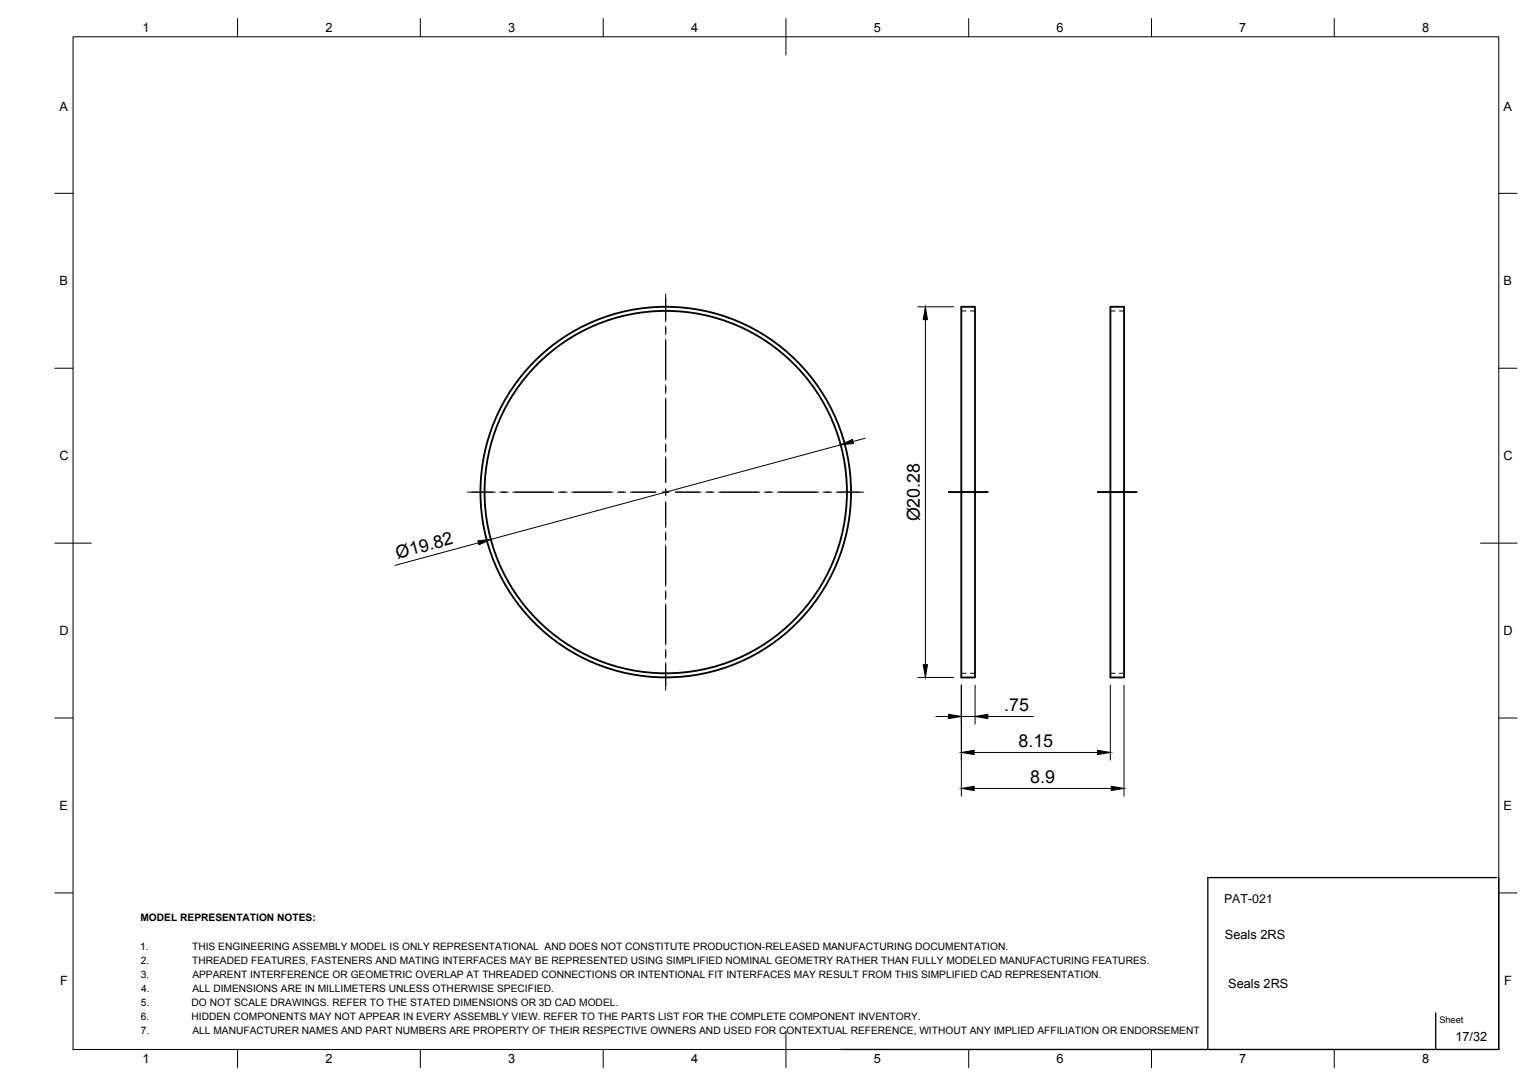
ISO-10303-21;
HEADER;
/* Generated by software containing ST-Developer
 * from STEP Tools, Inc. (www.steptools.com) 
 */

FILE_DESCRIPTION(
/* description */ ('Chain-less indexing wheel (Geneva) drive'),
/* implementation_level */ '2;1');

FILE_NAME(
/* name */ 'Seals 2RS.step',
/* time_stamp */ '2026-10-28T03:25:22-07:00',
/* author */ (''),
/* organization */ (''),
/* preprocessor_version */ 'ST-DEVELOPER v20.2',
/* originating_system */ 'Autodesk Translation Framework v15.17.0.0',
/* authorisation */ '');

FILE_SCHEMA (('AUTOMOTIVE_DESIGN { 1 0 10303 214 3 1 1 }'));
ENDSEC;

DATA;
#10=MECHANICAL_DESIGN_GEOMETRIC_PRESENTATION_REPRESENTATION('',(#321,#322),#10957);
#264=SHAPE_REPRESENTATION_RELATIONSHIP('SRR','None',#11078,#289);
#289=ADVANCED_BREP_SHAPE_REPRESENTATION('',(#353,#354),#10941);
#321=STYLED_ITEM('',(#11287),#353);
#322=STYLED_ITEM('',(#11287),#354);
#353=MANIFOLD_SOLID_BREP('Body1',#5718);
#354=MANIFOLD_SOLID_BREP('Body2',#5719);
#429=FACE_BOUND('',#1216,.T.);
#430=FACE_BOUND('',#1219,.T.);
#431=FACE_BOUND('',#1222,.T.);
#432=FACE_BOUND('',#1225,.T.);
#552=PLANE('',#6383);
#553=PLANE('',#6388);
#554=PLANE('',#6391);
#555=PLANE('',#6396);
#820=FACE_OUTER_BOUND('',#1215,.T.);
#821=FACE_OUTER_BOUND('',#1217,.T.);
#822=FACE_OUTER_BOUND('',#1218,.T.);
#823=FACE_OUTER_BOUND('',#1220,.T.);
#824=FACE_OUTER_BOUND('',#1221,.T.);
#825=FACE_OUTER_BOUND('',#1223,.T.);
#826=FACE_OUTER_BOUND('',#1224,.T.);
#827=FACE_OUTER_BOUND('',#1226,.T.);
#1215=EDGE_LOOP('',(#4487));
#1216=EDGE_LOOP('',(#4488));
#1217=EDGE_LOOP('',(#4489,#4490,#4491,#4492));
#1218=EDGE_LOOP('',(#4493));
#1219=EDGE_LOOP('',(#4494));
#1220=EDGE_LOOP('',(#4495,#4496,#4497,#4498));
#1221=EDGE_LOOP('',(#4499));
#1222=EDGE_LOOP('',(#4500));
#1223=EDGE_LOOP('',(#4501,#4502,#4503,#4504));
#1224=EDGE_LOOP('',(#4505));
#1225=EDGE_LOOP('',(#4506));
#1226=EDGE_LOOP('',(#4507,#4508,#4509,#4510));
#1583=LINE('',#9810,#1957);
#1584=LINE('',#9815,#1958);
#1585=LINE('',#9824,#1959);
#1586=LINE('',#9829,#1960);
#1957=VECTOR('',#7665,1.013815);
#1958=VECTOR('',#7672,0.991185);
#1959=VECTOR('',#7683,1.013815);
#1960=VECTOR('',#7690,0.991185);
#2361=CIRCLE('',#6384,1.013815);
#2362=CIRCLE('',#6385,0.991185);
#2363=CIRCLE('',#6387,1.013815);
#2364=CIRCLE('',#6389,0.991185);
#2365=CIRCLE('',#6392,1.013815);
#2366=CIRCLE('',#6393,0.991185);
#2367=CIRCLE('',#6395,1.013815);
#2368=CIRCLE('',#6397,0.991185);
#2749=VERTEX_POINT('',#9803);
#2750=VERTEX_POINT('',#9805);
#2751=VERTEX_POINT('',#9808);
#2752=VERTEX_POINT('',#9812);
#2753=VERTEX_POINT('',#9817);
#2754=VERTEX_POINT('',#9819);
#2755=VERTEX_POINT('',#9822);
#2756=VERTEX_POINT('',#9826);
#3369=EDGE_CURVE('',#2749,#2749,#2361,.T.);
#3370=EDGE_CURVE('',#2750,#2750,#2362,.T.);
#3371=EDGE_CURVE('',#2751,#2751,#2363,.T.);
#3372=EDGE_CURVE('',#2751,#2749,#1583,.T.);
#3373=EDGE_CURVE('',#2752,#2752,#2364,.T.);
#3374=EDGE_CURVE('',#2752,#2750,#1584,.T.);
#3375=EDGE_CURVE('',#2753,#2753,#2365,.T.);
#3376=EDGE_CURVE('',#2754,#2754,#2366,.T.);
#3377=EDGE_CURVE('',#2755,#2755,#2367,.T.);
#3378=EDGE_CURVE('',#2755,#2753,#1585,.T.);
#3379=EDGE_CURVE('',#2756,#2756,#2368,.T.);
#3380=EDGE_CURVE('',#2756,#2754,#1586,.T.);
#4487=ORIENTED_EDGE('',*,*,#3369,.F.);
#4488=ORIENTED_EDGE('',*,*,#3370,.T.);
#4489=ORIENTED_EDGE('',*,*,#3371,.F.);
#4490=ORIENTED_EDGE('',*,*,#3372,.T.);
#4491=ORIENTED_EDGE('',*,*,#3369,.T.);
#4492=ORIENTED_EDGE('',*,*,#3372,.F.);
#4493=ORIENTED_EDGE('',*,*,#3371,.T.);
#4494=ORIENTED_EDGE('',*,*,#3373,.F.);
#4495=ORIENTED_EDGE('',*,*,#3373,.T.);
#4496=ORIENTED_EDGE('',*,*,#3374,.T.);
#4497=ORIENTED_EDGE('',*,*,#3370,.F.);
#4498=ORIENTED_EDGE('',*,*,#3374,.F.);
#4499=ORIENTED_EDGE('',*,*,#3375,.F.);
#4500=ORIENTED_EDGE('',*,*,#3376,.T.);
#4501=ORIENTED_EDGE('',*,*,#3377,.F.);
#4502=ORIENTED_EDGE('',*,*,#3378,.T.);
#4503=ORIENTED_EDGE('',*,*,#3375,.T.);
#4504=ORIENTED_EDGE('',*,*,#3378,.F.);
#4505=ORIENTED_EDGE('',*,*,#3377,.T.);
#4506=ORIENTED_EDGE('',*,*,#3379,.F.);
#4507=ORIENTED_EDGE('',*,*,#3379,.T.);
#4508=ORIENTED_EDGE('',*,*,#3380,.T.);
#4509=ORIENTED_EDGE('',*,*,#3376,.F.);
#4510=ORIENTED_EDGE('',*,*,#3380,.F.);
#5305=CYLINDRICAL_SURFACE('',#6386,1.013815);
#5306=CYLINDRICAL_SURFACE('',#6390,0.991185);
#5307=CYLINDRICAL_SURFACE('',#6394,1.013815);
#5308=CYLINDRICAL_SURFACE('',#6398,0.991185);
#5534=ADVANCED_FACE('',(#820,#429),#552,.T.);
#5535=ADVANCED_FACE('',(#821),#5305,.T.);
#5536=ADVANCED_FACE('',(#822,#430),#553,.T.);
#5537=ADVANCED_FACE('',(#823),#5306,.F.);
#5538=ADVANCED_FACE('',(#824,#431),#554,.T.);
#5539=ADVANCED_FACE('',(#825),#5307,.T.);
#5540=ADVANCED_FACE('',(#826,#432),#555,.T.);
#5541=ADVANCED_FACE('',(#827),#5308,.F.);
#5718=CLOSED_SHELL('',(#5534,#5535,#5536,#5537));
#5719=CLOSED_SHELL('',(#5538,#5539,#5540,#5541));
#6382=AXIS2_PLACEMENT_3D('',#9801,#7653,#7654);
#6383=AXIS2_PLACEMENT_3D('',#9802,#7655,#7656);
#6384=AXIS2_PLACEMENT_3D('',#9804,#7657,#7658);
#6385=AXIS2_PLACEMENT_3D('',#9806,#7659,#7660);
#6386=AXIS2_PLACEMENT_3D('',#9807,#7661,#7662);
#6387=AXIS2_PLACEMENT_3D('',#9809,#7663,#7664);
#6388=AXIS2_PLACEMENT_3D('',#9811,#7666,#7667);
#6389=AXIS2_PLACEMENT_3D('',#9813,#7668,#7669);
#6390=AXIS2_PLACEMENT_3D('',#9814,#7670,#7671);
#6391=AXIS2_PLACEMENT_3D('',#9816,#7673,#7674);
#6392=AXIS2_PLACEMENT_3D('',#9818,#7675,#7676);
#6393=AXIS2_PLACEMENT_3D('',#9820,#7677,#7678);
#6394=AXIS2_PLACEMENT_3D('',#9821,#7679,#7680);
#6395=AXIS2_PLACEMENT_3D('',#9823,#7681,#7682);
#6396=AXIS2_PLACEMENT_3D('',#9825,#7684,#7685);
#6397=AXIS2_PLACEMENT_3D('',#9827,#7686,#7687);
#6398=AXIS2_PLACEMENT_3D('',#9828,#7688,#7689);
#7653=DIRECTION('axis',(0.,0.,1.));
#7654=DIRECTION('refdir',(1.,0.,0.));
#7655=DIRECTION('center_axis',(0.,1.,0.));
#7656=DIRECTION('ref_axis',(0.,0.,1.));
#7657=DIRECTION('center_axis',(0.,-1.,0.));
#7658=DIRECTION('ref_axis',(1.,0.,0.));
#7659=DIRECTION('center_axis',(0.,-1.,0.));
#7660=DIRECTION('ref_axis',(1.,0.,0.));
#7661=DIRECTION('center_axis',(0.,-1.,0.));
#7662=DIRECTION('ref_axis',(1.,0.,0.));
#7663=DIRECTION('center_axis',(0.,-1.,0.));
#7664=DIRECTION('ref_axis',(1.,0.,0.));
#7665=DIRECTION('',(0.,1.,0.));
#7666=DIRECTION('center_axis',(0.,-1.,0.));
#7667=DIRECTION('ref_axis',(0.,0.,-1.));
#7668=DIRECTION('center_axis',(0.,-1.,0.));
#7669=DIRECTION('ref_axis',(1.,0.,0.));
#7670=DIRECTION('center_axis',(0.,-1.,0.));
#7671=DIRECTION('ref_axis',(1.,0.,0.));
#7672=DIRECTION('',(0.,1.,0.));
#7673=DIRECTION('center_axis',(0.,1.,0.));
#7674=DIRECTION('ref_axis',(0.,0.,1.));
#7675=DIRECTION('center_axis',(0.,-1.,0.));
#7676=DIRECTION('ref_axis',(1.,0.,0.));
#7677=DIRECTION('center_axis',(0.,-1.,0.));
#7678=DIRECTION('ref_axis',(1.,0.,0.));
#7679=DIRECTION('center_axis',(0.,-1.,0.));
#7680=DIRECTION('ref_axis',(1.,0.,0.));
#7681=DIRECTION('center_axis',(0.,-1.,0.));
#7682=DIRECTION('ref_axis',(1.,0.,0.));
#7683=DIRECTION('',(0.,1.,0.));
#7684=DIRECTION('center_axis',(0.,-1.,0.));
#7685=DIRECTION('ref_axis',(0.,0.,-1.));
#7686=DIRECTION('center_axis',(0.,-1.,0.));
#7687=DIRECTION('ref_axis',(1.,0.,0.));
#7688=DIRECTION('center_axis',(0.,-1.,0.));
#7689=DIRECTION('ref_axis',(1.,0.,0.));
#7690=DIRECTION('',(0.,1.,0.));
#9801=CARTESIAN_POINT('',(0.,0.,0.));
#9802=CARTESIAN_POINT('Origin',(1.013815,0.445,0.));
#9803=CARTESIAN_POINT('',(-1.013815,0.445,-1.24156529467757E-16));
#9804=CARTESIAN_POINT('Origin',(0.,0.445,0.));
#9805=CARTESIAN_POINT('',(-0.991185,0.445,-1.21385153761287E-16));
#9806=CARTESIAN_POINT('Origin',(0.,0.445,0.));
#9807=CARTESIAN_POINT('Origin',(0.,0.4075,0.));
#9808=CARTESIAN_POINT('',(-1.013815,0.37,-1.24156529467757E-16));
#9809=CARTESIAN_POINT('Origin',(0.,0.37,0.));
#9810=CARTESIAN_POINT('',(-1.013815,0.4075,-1.24156529467757E-16));
#9811=CARTESIAN_POINT('Origin',(0.991185,0.37,0.));
#9812=CARTESIAN_POINT('',(-0.991185,0.37,-1.21385153761287E-16));
#9813=CARTESIAN_POINT('Origin',(0.,0.37,0.));
#9814=CARTESIAN_POINT('Origin',(0.,0.4075,0.));
#9815=CARTESIAN_POINT('',(-0.991185,0.4075,-1.21385153761287E-16));
#9816=CARTESIAN_POINT('Origin',(1.013815,-0.37,0.));
#9817=CARTESIAN_POINT('',(-1.013815,-0.37,-1.24156529467757E-16));
#9818=CARTESIAN_POINT('Origin',(0.,-0.37,0.));
#9819=CARTESIAN_POINT('',(-0.991185,-0.37,-1.21385153761287E-16));
#9820=CARTESIAN_POINT('Origin',(0.,-0.37,0.));
#9821=CARTESIAN_POINT('Origin',(0.,-0.4075,0.));
#9822=CARTESIAN_POINT('',(-1.013815,-0.445,-1.24156529467757E-16));
#9823=CARTESIAN_POINT('Origin',(0.,-0.445,0.));
#9824=CARTESIAN_POINT('',(-1.013815,-0.4075,-1.24156529467757E-16));
#9825=CARTESIAN_POINT('Origin',(0.991185,-0.445,0.));
#9826=CARTESIAN_POINT('',(-0.991185,-0.445,-1.21385153761287E-16));
#9827=CARTESIAN_POINT('Origin',(0.,-0.445,0.));
#9828=CARTESIAN_POINT('Origin',(0.,-0.4075,0.));
#9829=CARTESIAN_POINT('',(-0.991185,-0.4075,-1.21385153761287E-16));
#10910=UNCERTAINTY_MEASURE_WITH_UNIT(LENGTH_MEASURE(0.001),#10958,
'DISTANCE_ACCURACY_VALUE',
'Maximum model space distance between geometric entities at asserted c
onnectivities');
#10926=UNCERTAINTY_MEASURE_WITH_UNIT(LENGTH_MEASURE(0.001),#10958,
'DISTANCE_ACCURACY_VALUE',
'Maximum model space distance between geometric entities at asserted c
onnectivities');
#10941=(
GEOMETRIC_REPRESENTATION_CONTEXT(3)
GLOBAL_UNCERTAINTY_ASSIGNED_CONTEXT((#10910))
GLOBAL_UNIT_ASSIGNED_CONTEXT((#10958,#10960,#10961))
REPRESENTATION_CONTEXT('','3D')
);
#10957=(
GEOMETRIC_REPRESENTATION_CONTEXT(3)
GLOBAL_UNCERTAINTY_ASSIGNED_CONTEXT((#10926))
GLOBAL_UNIT_ASSIGNED_CONTEXT((#10958,#10960,#10961))
REPRESENTATION_CONTEXT('','3D')
);
#10958=(
LENGTH_UNIT()
NAMED_UNIT(*)
SI_UNIT(.CENTI.,.METRE.)
);
#10960=(
NAMED_UNIT(*)
PLANE_ANGLE_UNIT()
SI_UNIT($,.RADIAN.)
);
#10961=(
NAMED_UNIT(*)
SI_UNIT($,.STERADIAN.)
SOLID_ANGLE_UNIT()
);
#10976=SHAPE_DEFINITION_REPRESENTATION(#11006,#11078);
#11006=PRODUCT_DEFINITION_SHAPE('',$,#11109);
#11078=SHAPE_REPRESENTATION('',(#6382),#10941);
#11094=PRODUCT_DEFINITION_CONTEXT('part definition',#11186,'design');
#11109=PRODUCT_DEFINITION('Seals 2RS','Seals 2RS',#11139,#11094);
#11139=PRODUCT_DEFINITION_FORMATION('',$,#11202);
#11186=APPLICATION_CONTEXT(
'Core Data for Automotive Mechanical Design Process');
#11187=PRODUCT_CONTEXT('part definition',#11186,'mechanical');
#11202=PRODUCT('Seals 2RS','Seals 2RS','Seals 2RS',(#11187));
#11281=COLOUR_RGB('Grey',0.48,0.52,0.57);
#11282=FILL_AREA_STYLE_COLOUR('',#11281);
#11283=FILL_AREA_STYLE('',(#11282));
#11284=SURFACE_STYLE_FILL_AREA(#11283);
#11285=SURFACE_SIDE_STYLE('',(#11284));
#11286=SURFACE_STYLE_USAGE(.BOTH.,#11285);
#11287=PRESENTATION_STYLE_ASSIGNMENT((#11286));
ENDSEC;
END-ISO-10303-21;
